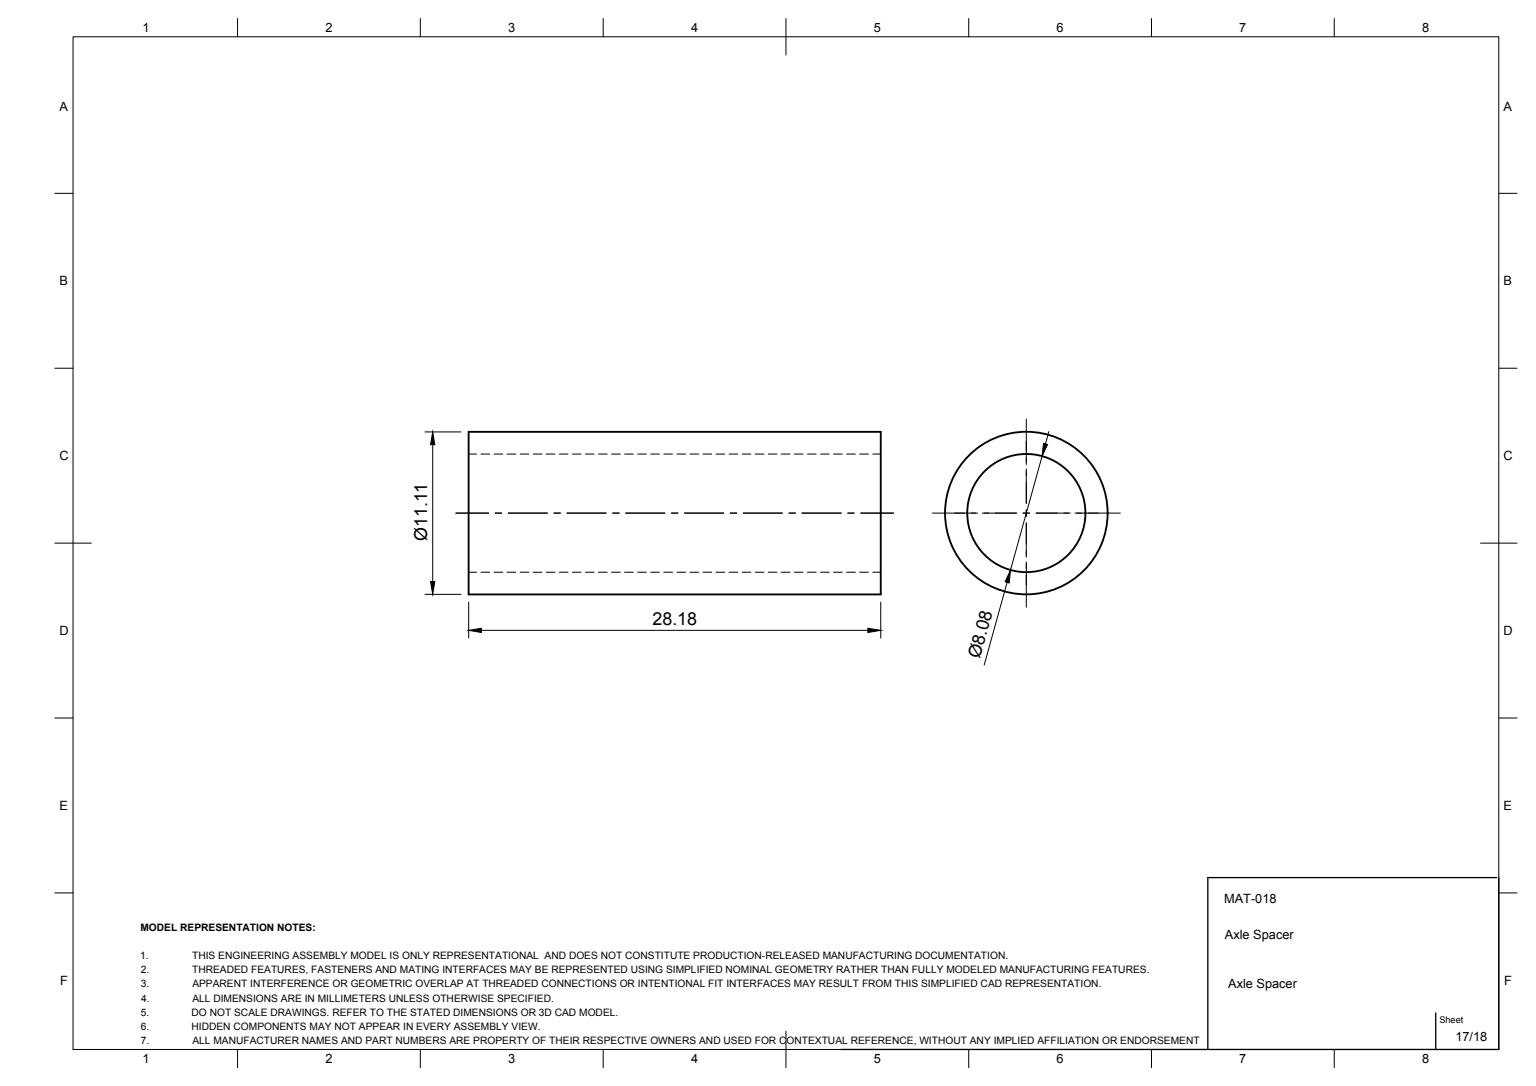
ISO-10303-21;
HEADER;
/* Generated by software containing ST-Developer
 * from STEP Tools, Inc. (www.steptools.com) 
 */

FILE_DESCRIPTION(
/* description */ ('STEP AP214'),
/* implementation_level */ '2;1');

FILE_NAME(
/* name */ 'Axle Spacer.step',
/* time_stamp */ '2026-11-14T06:16:09-08:00',
/* author */ (''),
/* organization */ (''),
/* preprocessor_version */ 'ST-DEVELOPER v20.2',
/* originating_system */ 'Autodesk Translation Framework v15.17.0.0',
/* authorisation */ '');

FILE_SCHEMA (('AUTOMOTIVE_DESIGN { 1 0 10303 214 3 1 1 }'));
ENDSEC;

DATA;
#10=MECHANICAL_DESIGN_GEOMETRIC_PRESENTATION_REPRESENTATION('',(#361),#18006);
#329=SHAPE_REPRESENTATION_RELATIONSHIP('SRR','None',#18087,#345);
#345=ADVANCED_BREP_SHAPE_REPRESENTATION('',(#377),#18004);
#361=STYLED_ITEM('',(#18171),#377);
#377=MANIFOLD_SOLID_BREP('Body1',#9570);
#498=FACE_BOUND('',#2105,.T.);
#499=FACE_BOUND('',#2107,.T.);
#837=PLANE('',#10824);
#838=PLANE('',#10825);
#1407=FACE_OUTER_BOUND('',#2102,.T.);
#1408=FACE_OUTER_BOUND('',#2103,.T.);
#1409=FACE_OUTER_BOUND('',#2104,.T.);
#1410=FACE_OUTER_BOUND('',#2106,.T.);
#2102=EDGE_LOOP('',(#8774,#8775,#8776,#8777));
#2103=EDGE_LOOP('',(#8778,#8779,#8780,#8781));
#2104=EDGE_LOOP('',(#8782));
#2105=EDGE_LOOP('',(#8783));
#2106=EDGE_LOOP('',(#8784));
#2107=EDGE_LOOP('',(#8785));
#2834=LINE('',#17911,#3558);
#2835=LINE('',#17917,#3559);
#3558=VECTOR('',#13721,4.0386);
#3559=VECTOR('',#13728,5.55625);
#4002=CIRCLE('',#10819,4.0386);
#4003=CIRCLE('',#10820,4.0386);
#4004=CIRCLE('',#10822,5.55625);
#4005=CIRCLE('',#10823,5.55625);
#4813=VERTEX_POINT('',#17908);
#4814=VERTEX_POINT('',#17910);
#4815=VERTEX_POINT('',#17914);
#4816=VERTEX_POINT('',#17916);
#6135=EDGE_CURVE('',#4813,#4813,#4002,.T.);
#6136=EDGE_CURVE('',#4813,#4814,#2834,.T.);
#6137=EDGE_CURVE('',#4814,#4814,#4003,.T.);
#6138=EDGE_CURVE('',#4815,#4815,#4004,.T.);
#6139=EDGE_CURVE('',#4815,#4816,#2835,.T.);
#6140=EDGE_CURVE('',#4816,#4816,#4005,.T.);
#8774=ORIENTED_EDGE('',*,*,#6135,.F.);
#8775=ORIENTED_EDGE('',*,*,#6136,.T.);
#8776=ORIENTED_EDGE('',*,*,#6137,.T.);
#8777=ORIENTED_EDGE('',*,*,#6136,.F.);
#8778=ORIENTED_EDGE('',*,*,#6138,.F.);
#8779=ORIENTED_EDGE('',*,*,#6139,.T.);
#8780=ORIENTED_EDGE('',*,*,#6140,.T.);
#8781=ORIENTED_EDGE('',*,*,#6139,.F.);
#8782=ORIENTED_EDGE('',*,*,#6138,.T.);
#8783=ORIENTED_EDGE('',*,*,#6137,.F.);
#8784=ORIENTED_EDGE('',*,*,#6140,.F.);
#8785=ORIENTED_EDGE('',*,*,#6135,.T.);
#8976=CYLINDRICAL_SURFACE('',#10818,4.0386);
#8977=CYLINDRICAL_SURFACE('',#10821,5.55625);
#9546=ADVANCED_FACE('',(#1407),#8976,.F.);
#9547=ADVANCED_FACE('',(#1408),#8977,.T.);
#9548=ADVANCED_FACE('',(#1409,#498),#837,.T.);
#9549=ADVANCED_FACE('',(#1410,#499),#838,.T.);
#9570=CLOSED_SHELL('',(#9546,#9547,#9548,#9549));
#10817=AXIS2_PLACEMENT_3D('',#17906,#13715,#13716);
#10818=AXIS2_PLACEMENT_3D('',#17907,#13717,#13718);
#10819=AXIS2_PLACEMENT_3D('',#17909,#13719,#13720);
#10820=AXIS2_PLACEMENT_3D('',#17912,#13722,#13723);
#10821=AXIS2_PLACEMENT_3D('',#17913,#13724,#13725);
#10822=AXIS2_PLACEMENT_3D('',#17915,#13726,#13727);
#10823=AXIS2_PLACEMENT_3D('',#17918,#13729,#13730);
#10824=AXIS2_PLACEMENT_3D('',#17919,#13731,#13732);
#10825=AXIS2_PLACEMENT_3D('',#17920,#13733,#13734);
#13715=DIRECTION('axis',(0.,0.,1.));
#13716=DIRECTION('refdir',(1.,0.,0.));
#13717=DIRECTION('center_axis',(0.,0.,-1.));
#13718=DIRECTION('ref_axis',(-1.,0.,0.));
#13719=DIRECTION('center_axis',(0.,0.,-1.));
#13720=DIRECTION('ref_axis',(-1.,0.,0.));
#13721=DIRECTION('',(0.,0.,-1.));
#13722=DIRECTION('center_axis',(0.,0.,-1.));
#13723=DIRECTION('ref_axis',(-1.,0.,0.));
#13724=DIRECTION('center_axis',(0.,0.,-1.));
#13725=DIRECTION('ref_axis',(-1.,0.,0.));
#13726=DIRECTION('center_axis',(0.,0.,-1.));
#13727=DIRECTION('ref_axis',(-1.,0.,0.));
#13728=DIRECTION('',(0.,0.,1.));
#13729=DIRECTION('center_axis',(0.,0.,-1.));
#13730=DIRECTION('ref_axis',(-1.,0.,0.));
#13731=DIRECTION('center_axis',(0.,0.,-1.));
#13732=DIRECTION('ref_axis',(0.,-1.,0.));
#13733=DIRECTION('center_axis',(0.,0.,1.));
#13734=DIRECTION('ref_axis',(1.,0.,0.));
#17906=CARTESIAN_POINT('',(0.,0.,0.));
#17907=CARTESIAN_POINT('Origin',(0.,0.,-14.08938));
#17908=CARTESIAN_POINT('',(4.0386,-4.9458585630365E-16,14.08938));
#17909=CARTESIAN_POINT('Origin',(0.,0.,14.08938));
#17910=CARTESIAN_POINT('',(4.0386,-4.9458585630365E-16,-14.08938));
#17911=CARTESIAN_POINT('',(4.0386,-4.9458585630365E-16,-14.08938));
#17912=CARTESIAN_POINT('Origin',(0.,0.,-14.08938));
#17913=CARTESIAN_POINT('Origin',(0.,0.,-14.08938));
#17914=CARTESIAN_POINT('',(5.55625,-6.80444377776248E-16,-14.08938));
#17915=CARTESIAN_POINT('Origin',(0.,0.,-14.08938));
#17916=CARTESIAN_POINT('',(5.55625,-6.80444377776248E-16,14.08938));
#17917=CARTESIAN_POINT('',(5.55625,-6.80444377776248E-16,-14.08938));
#17918=CARTESIAN_POINT('Origin',(0.,0.,14.08938));
#17919=CARTESIAN_POINT('Origin',(0.,4.0386,-14.08938));
#17920=CARTESIAN_POINT('Origin',(0.,5.55625,14.08938));
#17984=UNCERTAINTY_MEASURE_WITH_UNIT(LENGTH_MEASURE(0.01),#18007,
'DISTANCE_ACCURACY_VALUE',
'Maximum model space distance between geometric entities at asserted c
onnectivities');
#17986=UNCERTAINTY_MEASURE_WITH_UNIT(LENGTH_MEASURE(0.01),#18007,
'DISTANCE_ACCURACY_VALUE',
'Maximum model space distance between geometric entities at asserted c
onnectivities');
#18004=(
GEOMETRIC_REPRESENTATION_CONTEXT(3)
GLOBAL_UNCERTAINTY_ASSIGNED_CONTEXT((#17984))
GLOBAL_UNIT_ASSIGNED_CONTEXT((#18007,#18009,#18010))
REPRESENTATION_CONTEXT('','3D')
);
#18006=(
GEOMETRIC_REPRESENTATION_CONTEXT(3)
GLOBAL_UNCERTAINTY_ASSIGNED_CONTEXT((#17986))
GLOBAL_UNIT_ASSIGNED_CONTEXT((#18007,#18009,#18010))
REPRESENTATION_CONTEXT('','3D')
);
#18007=(
LENGTH_UNIT()
NAMED_UNIT(*)
SI_UNIT(.MILLI.,.METRE.)
);
#18009=(
NAMED_UNIT(*)
PLANE_ANGLE_UNIT()
SI_UNIT($,.RADIAN.)
);
#18010=(
NAMED_UNIT(*)
SI_UNIT($,.STERADIAN.)
SOLID_ANGLE_UNIT()
);
#18028=SHAPE_DEFINITION_REPRESENTATION(#18047,#18087);
#18047=PRODUCT_DEFINITION_SHAPE('',$,#18107);
#18087=SHAPE_REPRESENTATION('',(#10817),#18004);
#18089=PRODUCT_DEFINITION_CONTEXT('part definition',#18148,'design');
#18107=PRODUCT_DEFINITION('Axle Spacer','Axle Spacer',#18126,#18089);
#18126=PRODUCT_DEFINITION_FORMATION('',$,#18167);
#18148=APPLICATION_CONTEXT(
'Core Data for Automotive Mechanical Design Process');
#18149=PRODUCT_CONTEXT('part definition',#18148,'mechanical');
#18167=PRODUCT('Axle Spacer','Axle Spacer',$,(#18149));
#18171=PRESENTATION_STYLE_ASSIGNMENT((#18175));
#18175=SURFACE_STYLE_USAGE(.BOTH.,#18179);
#18179=SURFACE_SIDE_STYLE('',(#18183));
#18183=SURFACE_STYLE_FILL_AREA(#18187);
#18187=FILL_AREA_STYLE('Opaque(61,176,222)',(#18191));
#18191=FILL_AREA_STYLE_COLOUR('Opaque(61,176,222)',#18195);
#18195=COLOUR_RGB('Opaque(61,176,222)',0.23921568627451,0.690196078431373,
0.870588235294118);
ENDSEC;
END-ISO-10303-21;
